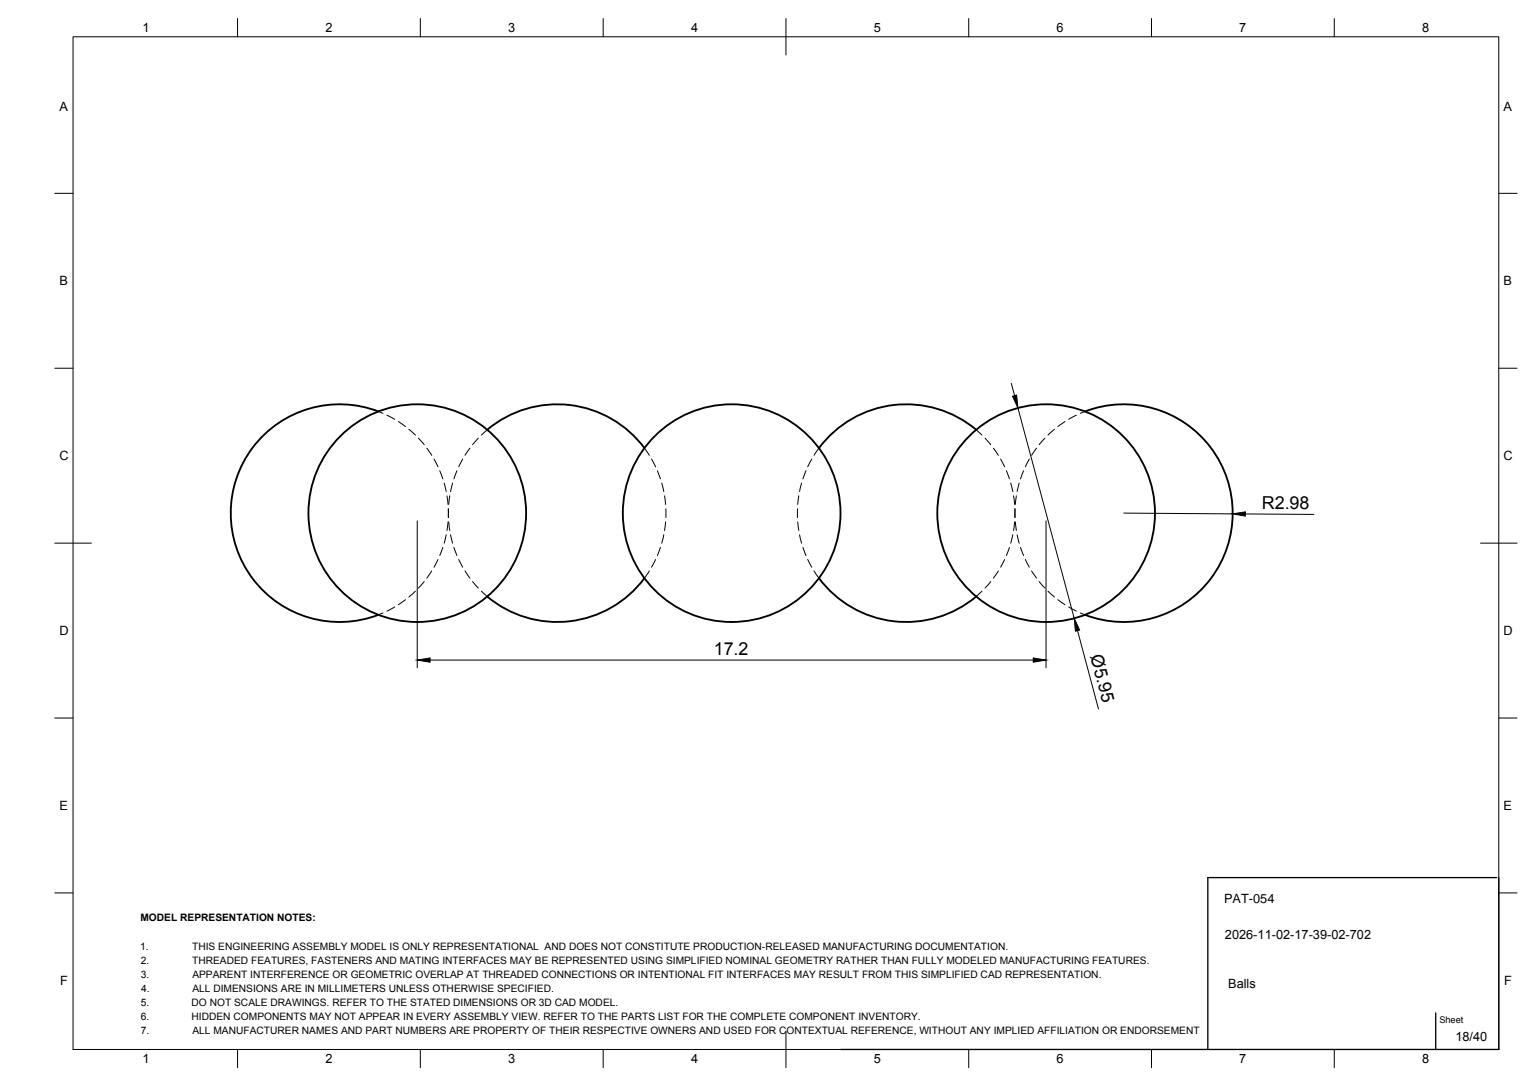
ISO-10303-21;
HEADER;
/* Generated by software containing ST-Developer
 * from STEP Tools, Inc. (www.steptools.com) 
 */

FILE_DESCRIPTION(
/* description */ ('PAT-054'),
/* implementation_level */ '2;1');

FILE_NAME(
/* name */ 'Balls.step',
/* time_stamp */ '2026-10-29T16:38:13-07:00',
/* author */ (''),
/* organization */ (''),
/* preprocessor_version */ 'ST-DEVELOPER v20.2',
/* originating_system */ 'Autodesk Translation Framework v15.17.0.0',
/* authorisation */ '');

FILE_SCHEMA (('AUTOMOTIVE_DESIGN { 1 0 10303 214 3 1 1 }'));
ENDSEC;

DATA;
#10=MECHANICAL_DESIGN_GEOMETRIC_PRESENTATION_REPRESENTATION('',(#910,#911,#912,#913,#914,#915,#916),#33981);
#747=SPHERICAL_SURFACE('',#13913,0.29765);
#748=SPHERICAL_SURFACE('',#13915,0.29765);
#749=SPHERICAL_SURFACE('',#13917,0.29765);
#750=SPHERICAL_SURFACE('',#13919,0.29765);
#751=SPHERICAL_SURFACE('',#13921,0.29765);
#752=SPHERICAL_SURFACE('',#13923,0.29765);
#753=SPHERICAL_SURFACE('',#13925,0.29765);
#822=SHAPE_REPRESENTATION_RELATIONSHIP('SRR','None',#34196,#866);
#866=ADVANCED_BREP_SHAPE_REPRESENTATION('',(#969,#970,#971,#972,#973,#974,
#975),#33944);
#910=STYLED_ITEM('',(#34517),#969);
#911=STYLED_ITEM('',(#34517),#970);
#912=STYLED_ITEM('',(#34517),#971);
#913=STYLED_ITEM('',(#34517),#972);
#914=STYLED_ITEM('',(#34517),#973);
#915=STYLED_ITEM('',(#34517),#974);
#916=STYLED_ITEM('',(#34517),#975);
#969=MANIFOLD_SOLID_BREP('Body1',#13021);
#970=MANIFOLD_SOLID_BREP('Body2',#13022);
#971=MANIFOLD_SOLID_BREP('Body3',#13023);
#972=MANIFOLD_SOLID_BREP('Body4',#13024);
#973=MANIFOLD_SOLID_BREP('Body5',#13025);
#974=MANIFOLD_SOLID_BREP('Body6',#13026);
#975=MANIFOLD_SOLID_BREP('Body7',#13027);
#1744=FACE_OUTER_BOUND('',#2587,.T.);
#1745=FACE_OUTER_BOUND('',#2588,.T.);
#1746=FACE_OUTER_BOUND('',#2589,.T.);
#1747=FACE_OUTER_BOUND('',#2590,.T.);
#1748=FACE_OUTER_BOUND('',#2591,.T.);
#1749=FACE_OUTER_BOUND('',#2592,.T.);
#1750=FACE_OUTER_BOUND('',#2593,.T.);
#2587=EDGE_LOOP('',(#9291,#9292));
#2588=EDGE_LOOP('',(#9293,#9294));
#2589=EDGE_LOOP('',(#9295,#9296));
#2590=EDGE_LOOP('',(#9297,#9298));
#2591=EDGE_LOOP('',(#9299,#9300));
#2592=EDGE_LOOP('',(#9301,#9302));
#2593=EDGE_LOOP('',(#9303,#9304));
#5275=CIRCLE('',#13914,0.29765);
#5276=CIRCLE('',#13916,0.29765);
#5277=CIRCLE('',#13918,0.29765);
#5278=CIRCLE('',#13920,0.29765);
#5279=CIRCLE('',#13922,0.29765);
#5280=CIRCLE('',#13924,0.29765);
#5281=CIRCLE('',#13926,0.29765);
#5836=VERTEX_POINT('',#19338);
#5837=VERTEX_POINT('',#19339);
#5838=VERTEX_POINT('',#19342);
#5839=VERTEX_POINT('',#19343);
#5840=VERTEX_POINT('',#19346);
#5841=VERTEX_POINT('',#19347);
#5842=VERTEX_POINT('',#19350);
#5843=VERTEX_POINT('',#19351);
#5844=VERTEX_POINT('',#19354);
#5845=VERTEX_POINT('',#19355);
#5846=VERTEX_POINT('',#19358);
#5847=VERTEX_POINT('',#19359);
#5848=VERTEX_POINT('',#19362);
#5849=VERTEX_POINT('',#19363);
#7145=EDGE_CURVE('',#5836,#5837,#5275,.T.);
#7146=EDGE_CURVE('',#5838,#5839,#5276,.T.);
#7147=EDGE_CURVE('',#5840,#5841,#5277,.T.);
#7148=EDGE_CURVE('',#5842,#5843,#5278,.T.);
#7149=EDGE_CURVE('',#5844,#5845,#5279,.T.);
#7150=EDGE_CURVE('',#5846,#5847,#5280,.T.);
#7151=EDGE_CURVE('',#5848,#5849,#5281,.T.);
#9291=ORIENTED_EDGE('',*,*,#7145,.T.);
#9292=ORIENTED_EDGE('',*,*,#7145,.F.);
#9293=ORIENTED_EDGE('',*,*,#7146,.T.);
#9294=ORIENTED_EDGE('',*,*,#7146,.F.);
#9295=ORIENTED_EDGE('',*,*,#7147,.T.);
#9296=ORIENTED_EDGE('',*,*,#7147,.F.);
#9297=ORIENTED_EDGE('',*,*,#7148,.T.);
#9298=ORIENTED_EDGE('',*,*,#7148,.F.);
#9299=ORIENTED_EDGE('',*,*,#7149,.T.);
#9300=ORIENTED_EDGE('',*,*,#7149,.F.);
#9301=ORIENTED_EDGE('',*,*,#7150,.T.);
#9302=ORIENTED_EDGE('',*,*,#7150,.F.);
#9303=ORIENTED_EDGE('',*,*,#7151,.T.);
#9304=ORIENTED_EDGE('',*,*,#7151,.F.);
#12456=ADVANCED_FACE('',(#1744),#747,.T.);
#12457=ADVANCED_FACE('',(#1745),#748,.T.);
#12458=ADVANCED_FACE('',(#1746),#749,.T.);
#12459=ADVANCED_FACE('',(#1747),#750,.T.);
#12460=ADVANCED_FACE('',(#1748),#751,.T.);
#12461=ADVANCED_FACE('',(#1749),#752,.T.);
#12462=ADVANCED_FACE('',(#1750),#753,.T.);
#13021=CLOSED_SHELL('',(#12456));
#13022=CLOSED_SHELL('',(#12457));
#13023=CLOSED_SHELL('',(#12458));
#13024=CLOSED_SHELL('',(#12459));
#13025=CLOSED_SHELL('',(#12460));
#13026=CLOSED_SHELL('',(#12461));
#13027=CLOSED_SHELL('',(#12462));
#13912=AXIS2_PLACEMENT_3D('',#19336,#15827,#15828);
#13913=AXIS2_PLACEMENT_3D('',#19337,#15829,#15830);
#13914=AXIS2_PLACEMENT_3D('',#19340,#15831,#15832);
#13915=AXIS2_PLACEMENT_3D('',#19341,#15833,#15834);
#13916=AXIS2_PLACEMENT_3D('',#19344,#15835,#15836);
#13917=AXIS2_PLACEMENT_3D('',#19345,#15837,#15838);
#13918=AXIS2_PLACEMENT_3D('',#19348,#15839,#15840);
#13919=AXIS2_PLACEMENT_3D('',#19349,#15841,#15842);
#13920=AXIS2_PLACEMENT_3D('',#19352,#15843,#15844);
#13921=AXIS2_PLACEMENT_3D('',#19353,#15845,#15846);
#13922=AXIS2_PLACEMENT_3D('',#19356,#15847,#15848);
#13923=AXIS2_PLACEMENT_3D('',#19357,#15849,#15850);
#13924=AXIS2_PLACEMENT_3D('',#19360,#15851,#15852);
#13925=AXIS2_PLACEMENT_3D('',#19361,#15853,#15854);
#13926=AXIS2_PLACEMENT_3D('',#19364,#15855,#15856);
#15827=DIRECTION('axis',(0.,0.,1.));
#15828=DIRECTION('refdir',(1.,0.,0.));
#15829=DIRECTION('center_axis',(0.,0.,1.));
#15830=DIRECTION('ref_axis',(1.,0.,0.));
#15831=DIRECTION('center_axis',(1.22464679914735E-16,-1.,0.));
#15832=DIRECTION('ref_axis',(-1.,-1.22464679914735E-16,0.));
#15833=DIRECTION('center_axis',(0.78183148246803,0.,0.623489801858733));
#15834=DIRECTION('ref_axis',(0.623489801858734,0.,-0.78183148246803));
#15835=DIRECTION('center_axis',(7.63554790147315E-17,-1.,-9.57467422477103E-17));
#15836=DIRECTION('ref_axis',(-0.623489801858734,-1.22464679914735E-16,0.78183148246803));
#15837=DIRECTION('center_axis',(0.974927912181824,0.,-0.222520933956314));
#15838=DIRECTION('ref_axis',(-0.222520933956314,0.,-0.974927912181824));
#15839=DIRECTION('center_axis',(-2.7250954951288E-17,-1.,-1.19394234705288E-16));
#15840=DIRECTION('ref_axis',(0.222520933956314,-1.22464679914735E-16,0.974927912181824));
#15841=DIRECTION('center_axis',(0.433883739117558,0.,-0.900968867902419));
#15842=DIRECTION('ref_axis',(-0.900968867902419,0.,-0.433883739117558));
#15843=DIRECTION('center_axis',(-1.10336864020811E-16,-1.,-5.31354332312403E-17));
#15844=DIRECTION('ref_axis',(0.900968867902419,-1.22464679914735E-16,0.433883739117558));
#15845=DIRECTION('center_axis',(-0.433883739117558,0.,-0.900968867902419));
#15846=DIRECTION('ref_axis',(-0.900968867902419,0.,0.433883739117558));
#15847=DIRECTION('center_axis',(-1.10336864020811E-16,-1.,5.31354332312403E-17));
#15848=DIRECTION('ref_axis',(0.900968867902419,-1.22464679914735E-16,-0.433883739117558));
#15849=DIRECTION('center_axis',(-0.974927912181824,0.,-0.222520933956314));
#15850=DIRECTION('ref_axis',(-0.222520933956315,0.,0.974927912181824));
#15851=DIRECTION('center_axis',(-2.7250954951288E-17,-1.,1.19394234705288E-16));
#15852=DIRECTION('ref_axis',(0.222520933956315,-1.22464679914735E-16,-0.974927912181824));
#15853=DIRECTION('center_axis',(-0.78183148246803,0.,0.623489801858734));
#15854=DIRECTION('ref_axis',(0.623489801858733,0.,0.78183148246803));
#15855=DIRECTION('center_axis',(7.63554790147315E-17,-1.,9.57467422477103E-17));
#15856=DIRECTION('ref_axis',(-0.623489801858733,-1.22464679914735E-16,-0.78183148246803));
#19336=CARTESIAN_POINT('',(0.,0.,0.));
#19337=CARTESIAN_POINT('Origin',(1.1,0.,0.));
#19338=CARTESIAN_POINT('',(1.1,-2.23201749654651E-33,0.29765));
#19339=CARTESIAN_POINT('',(1.1,-2.23201749654651E-33,-0.29765));
#19340=CARTESIAN_POINT('Origin',(1.1,0.,0.));
#19341=CARTESIAN_POINT('Origin',(0.685838782044607,0.,-0.860014630714833));
#19342=CARTESIAN_POINT('',(0.918550922801216,-5.31350540756609E-33,-0.674432891191581));
#19343=CARTESIAN_POINT('',(0.453126641287998,8.49470414473068E-34,-1.04559637023808));
#19344=CARTESIAN_POINT('Origin',(0.685838782044607,0.,-0.860014630714833));
#19345=CARTESIAN_POINT('Origin',(-0.244773027351946,0.,-1.07242070340001));
#19346=CARTESIAN_POINT('',(0.0454142657089739,-2.23201749654651E-33,-1.1386540593921));
#19347=CARTESIAN_POINT('',(-0.534960320412865,-2.23201749654651E-33,-1.00618734740791));
#19348=CARTESIAN_POINT('Origin',(-0.244773027351946,0.,-1.07242070340001));
#19349=CARTESIAN_POINT('Origin',(-0.991065754692661,0.,-0.477272113029314));
#19350=CARTESIAN_POINT('',(-0.86192025974432,8.49470414473067E-34,-0.745445496560469));
#19351=CARTESIAN_POINT('',(-1.120211249641,-5.31350540756609E-33,-0.209098729498159));
#19352=CARTESIAN_POINT('Origin',(-0.991065754692661,0.,-0.477272113029314));
#19353=CARTESIAN_POINT('Origin',(-0.991065754692661,0.,0.477272113029314));
#19354=CARTESIAN_POINT('',(-1.120211249641,-2.23201749654651E-33,0.209098729498159));
#19355=CARTESIAN_POINT('',(-0.86192025974432,-2.23201749654651E-33,0.745445496560469));
#19356=CARTESIAN_POINT('Origin',(-0.991065754692661,0.,0.477272113029314));
#19357=CARTESIAN_POINT('Origin',(-0.244773027351946,0.,1.07242070340001));
#19358=CARTESIAN_POINT('',(-0.534960320412866,-2.23201749654651E-33,1.00618734740791));
#19359=CARTESIAN_POINT('',(0.0454142657089737,-2.23201749654651E-33,1.1386540593921));
#19360=CARTESIAN_POINT('Origin',(-0.244773027351946,0.,1.07242070340001));
#19361=CARTESIAN_POINT('Origin',(0.685838782044607,0.,0.860014630714833));
#19362=CARTESIAN_POINT('',(0.453126641287998,-2.23201749654651E-33,1.04559637023808));
#19363=CARTESIAN_POINT('',(0.918550922801216,-2.23201749654651E-33,0.674432891191581));
#19364=CARTESIAN_POINT('Origin',(0.685838782044607,0.,0.860014630714833));
#33892=UNCERTAINTY_MEASURE_WITH_UNIT(LENGTH_MEASURE(0.001),#33982,
'DISTANCE_ACCURACY_VALUE',
'Maximum model space distance between geometric entities at asserted c
onnectivities');
#33929=UNCERTAINTY_MEASURE_WITH_UNIT(LENGTH_MEASURE(0.001),#33982,
'DISTANCE_ACCURACY_VALUE',
'Maximum model space distance between geometric entities at asserted c
onnectivities');
#33944=(
GEOMETRIC_REPRESENTATION_CONTEXT(3)
GLOBAL_UNCERTAINTY_ASSIGNED_CONTEXT((#33892))
GLOBAL_UNIT_ASSIGNED_CONTEXT((#33982,#33984,#33985))
REPRESENTATION_CONTEXT('','3D')
);
#33981=(
GEOMETRIC_REPRESENTATION_CONTEXT(3)
GLOBAL_UNCERTAINTY_ASSIGNED_CONTEXT((#33929))
GLOBAL_UNIT_ASSIGNED_CONTEXT((#33982,#33984,#33985))
REPRESENTATION_CONTEXT('','3D')
);
#33982=(
LENGTH_UNIT()
NAMED_UNIT(*)
SI_UNIT(.CENTI.,.METRE.)
);
#33984=(
NAMED_UNIT(*)
PLANE_ANGLE_UNIT()
SI_UNIT($,.RADIAN.)
);
#33985=(
NAMED_UNIT(*)
SI_UNIT($,.STERADIAN.)
SOLID_ANGLE_UNIT()
);
#34000=SHAPE_DEFINITION_REPRESENTATION(#34051,#34196);
#34051=PRODUCT_DEFINITION_SHAPE('',$,#34248);
#34196=SHAPE_REPRESENTATION('',(#13912),#33944);
#34233=PRODUCT_DEFINITION_CONTEXT('part definition',#34388,'design');
#34248=PRODUCT_DEFINITION('Balls','Balls',#34299,#34233);
#34299=PRODUCT_DEFINITION_FORMATION('',$,#34404);
#34388=APPLICATION_CONTEXT(
'Core Data for Automotive Mechanical Design Process');
#34389=PRODUCT_CONTEXT('part definition',#34388,'mechanical');
#34404=PRODUCT('Balls','Balls','Balls',(#34389));
#34511=COLOUR_RGB('Grey',0.48,0.52,0.57);
#34512=FILL_AREA_STYLE_COLOUR('',#34511);
#34513=FILL_AREA_STYLE('',(#34512));
#34514=SURFACE_STYLE_FILL_AREA(#34513);
#34515=SURFACE_SIDE_STYLE('',(#34514));
#34516=SURFACE_STYLE_USAGE(.BOTH.,#34515);
#34517=PRESENTATION_STYLE_ASSIGNMENT((#34516));
ENDSEC;
END-ISO-10303-21;
